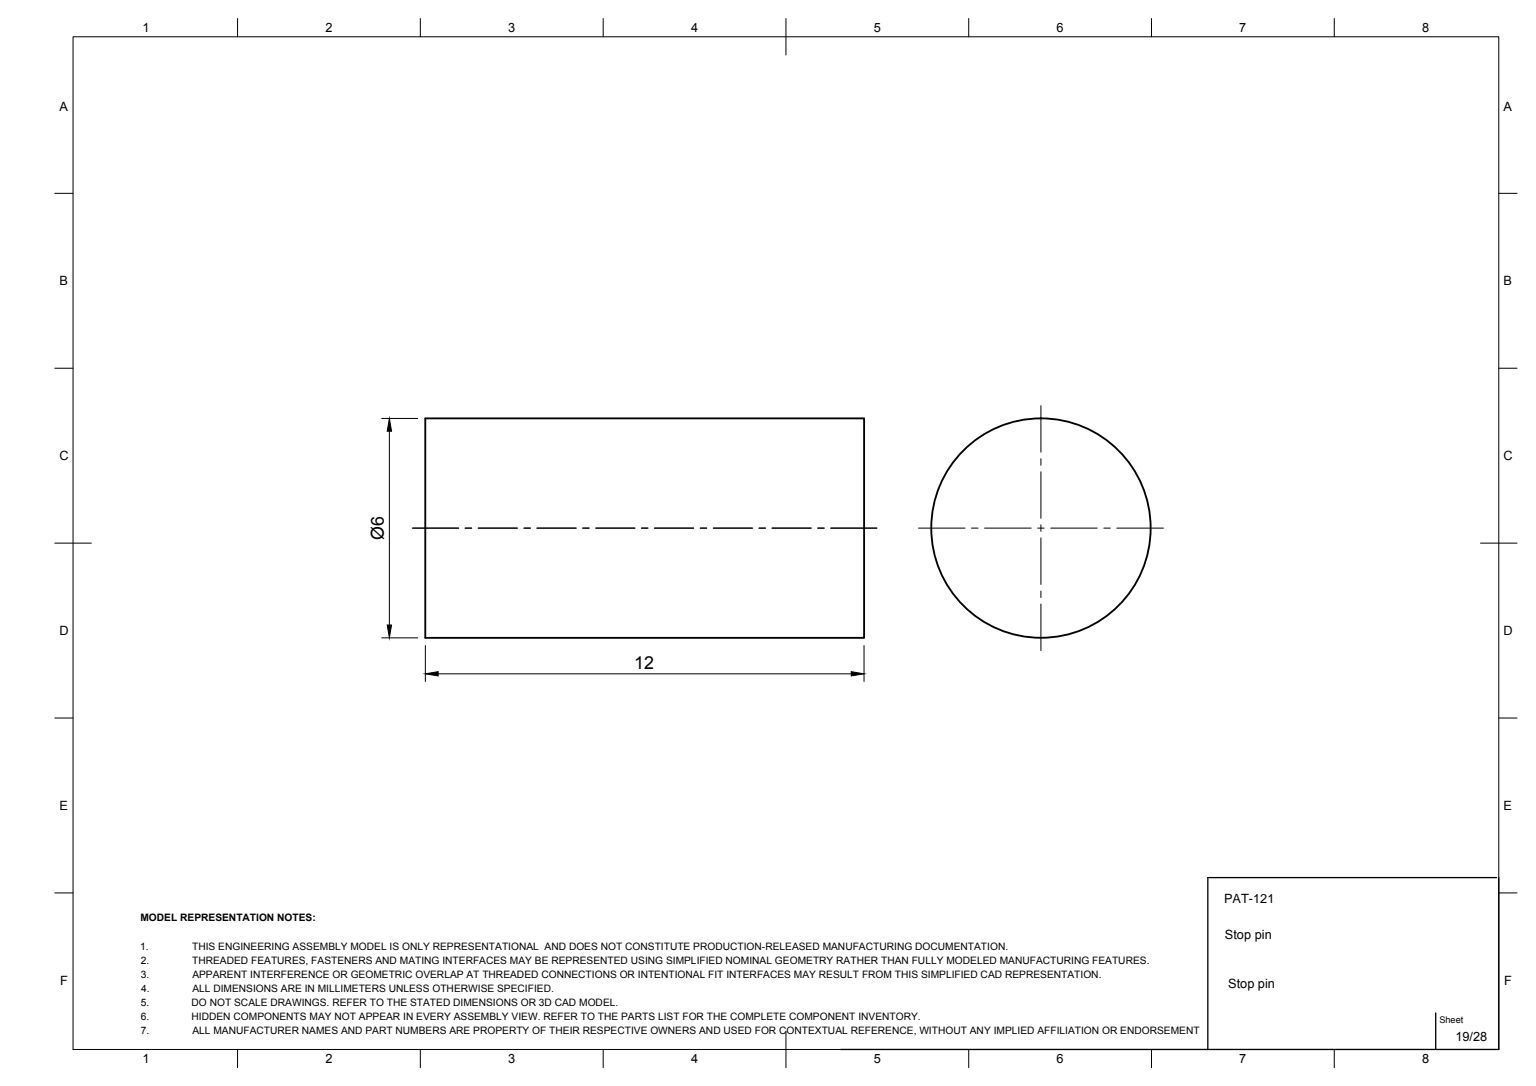
ISO-10303-21;
HEADER;
/* Generated by software containing ST-Developer
 * from STEP Tools, Inc. (www.steptools.com) 
 */

FILE_DESCRIPTION(
/* description */ ('Wall-mounted air drop station'),
/* implementation_level */ '2;1');

FILE_NAME(
/* name */ 'Stop pin.step',
/* time_stamp */ '2026-10-28T22:16:19-07:00',
/* author */ (''),
/* organization */ (''),
/* preprocessor_version */ 'ST-DEVELOPER v20.2',
/* originating_system */ 'Autodesk Translation Framework v15.17.0.0',
/* authorisation */ '');

FILE_SCHEMA (('AUTOMOTIVE_DESIGN { 1 0 10303 214 3 1 1 }'));
ENDSEC;

DATA;
#10=MECHANICAL_DESIGN_GEOMETRIC_PRESENTATION_REPRESENTATION('',(#363),#10517);
#305=SHAPE_REPRESENTATION_RELATIONSHIP('SRR','None',#10662,#334);
#334=ADVANCED_BREP_SHAPE_REPRESENTATION('',(#390),#10506);
#363=STYLED_ITEM('',(#10874),#390);
#390=MANIFOLD_SOLID_BREP('Body1',#5904);
#674=PLANE('',#6683);
#675=PLANE('',#6684);
#999=FACE_OUTER_BOUND('',#1460,.T.);
#1000=FACE_OUTER_BOUND('',#1461,.T.);
#1001=FACE_OUTER_BOUND('',#1462,.T.);
#1460=EDGE_LOOP('',(#4981,#4982,#4983,#4984));
#1461=EDGE_LOOP('',(#4985));
#1462=EDGE_LOOP('',(#4986));
#1905=LINE('',#9896,#2369);
#2369=VECTOR('',#8131,0.3);
#2699=CIRCLE('',#6681,0.3);
#2700=CIRCLE('',#6682,0.3);
#3097=VERTEX_POINT('',#9893);
#3098=VERTEX_POINT('',#9895);
#3748=EDGE_CURVE('',#3097,#3097,#2699,.T.);
#3749=EDGE_CURVE('',#3097,#3098,#1905,.T.);
#3750=EDGE_CURVE('',#3098,#3098,#2700,.T.);
#4981=ORIENTED_EDGE('',*,*,#3748,.F.);
#4982=ORIENTED_EDGE('',*,*,#3749,.T.);
#4983=ORIENTED_EDGE('',*,*,#3750,.T.);
#4984=ORIENTED_EDGE('',*,*,#3749,.F.);
#4985=ORIENTED_EDGE('',*,*,#3748,.T.);
#4986=ORIENTED_EDGE('',*,*,#3750,.F.);
#5508=CYLINDRICAL_SURFACE('',#6680,0.3);
#5772=ADVANCED_FACE('',(#999),#5508,.T.);
#5773=ADVANCED_FACE('',(#1000),#674,.T.);
#5774=ADVANCED_FACE('',(#1001),#675,.F.);
#5904=CLOSED_SHELL('',(#5772,#5773,#5774));
#6679=AXIS2_PLACEMENT_3D('',#9891,#8125,#8126);
#6680=AXIS2_PLACEMENT_3D('',#9892,#8127,#8128);
#6681=AXIS2_PLACEMENT_3D('',#9894,#8129,#8130);
#6682=AXIS2_PLACEMENT_3D('',#9897,#8132,#8133);
#6683=AXIS2_PLACEMENT_3D('',#9898,#8134,#8135);
#6684=AXIS2_PLACEMENT_3D('',#9899,#8136,#8137);
#8125=DIRECTION('axis',(0.,0.,1.));
#8126=DIRECTION('refdir',(1.,0.,0.));
#8127=DIRECTION('center_axis',(0.,0.,1.));
#8128=DIRECTION('ref_axis',(1.,0.,0.));
#8129=DIRECTION('center_axis',(0.,0.,1.));
#8130=DIRECTION('ref_axis',(1.,0.,0.));
#8131=DIRECTION('',(0.,0.,-1.));
#8132=DIRECTION('center_axis',(0.,0.,1.));
#8133=DIRECTION('ref_axis',(1.,0.,0.));
#8134=DIRECTION('center_axis',(0.,0.,1.));
#8135=DIRECTION('ref_axis',(1.,0.,0.));
#8136=DIRECTION('center_axis',(0.,0.,1.));
#8137=DIRECTION('ref_axis',(1.,0.,0.));
#9891=CARTESIAN_POINT('',(0.,0.,0.));
#9892=CARTESIAN_POINT('Origin',(3.,1.1,8.2));
#9893=CARTESIAN_POINT('',(2.7,1.1,9.4));
#9894=CARTESIAN_POINT('Origin',(3.,1.1,9.4));
#9895=CARTESIAN_POINT('',(2.7,1.1,8.2));
#9896=CARTESIAN_POINT('',(2.7,1.1,8.2));
#9897=CARTESIAN_POINT('Origin',(3.,1.1,8.2));
#9898=CARTESIAN_POINT('Origin',(3.,1.1,9.4));
#9899=CARTESIAN_POINT('Origin',(3.,1.1,8.2));
#10473=UNCERTAINTY_MEASURE_WITH_UNIT(LENGTH_MEASURE(0.001),#10518,
'DISTANCE_ACCURACY_VALUE',
'Maximum model space distance between geometric entities at asserted c
onnectivities');
#10484=UNCERTAINTY_MEASURE_WITH_UNIT(LENGTH_MEASURE(0.001),#10518,
'DISTANCE_ACCURACY_VALUE',
'Maximum model space distance between geometric entities at asserted c
onnectivities');
#10506=(
GEOMETRIC_REPRESENTATION_CONTEXT(3)
GLOBAL_UNCERTAINTY_ASSIGNED_CONTEXT((#10473))
GLOBAL_UNIT_ASSIGNED_CONTEXT((#10518,#10520,#10521))
REPRESENTATION_CONTEXT('','3D')
);
#10517=(
GEOMETRIC_REPRESENTATION_CONTEXT(3)
GLOBAL_UNCERTAINTY_ASSIGNED_CONTEXT((#10484))
GLOBAL_UNIT_ASSIGNED_CONTEXT((#10518,#10520,#10521))
REPRESENTATION_CONTEXT('','3D')
);
#10518=(
LENGTH_UNIT()
NAMED_UNIT(*)
SI_UNIT(.CENTI.,.METRE.)
);
#10520=(
NAMED_UNIT(*)
PLANE_ANGLE_UNIT()
SI_UNIT($,.RADIAN.)
);
#10521=(
NAMED_UNIT(*)
SI_UNIT($,.STERADIAN.)
SOLID_ANGLE_UNIT()
);
#10543=SHAPE_DEFINITION_REPRESENTATION(#10575,#10662);
#10575=PRODUCT_DEFINITION_SHAPE('',$,#10695);
#10662=SHAPE_REPRESENTATION('',(#6679),#10506);
#10673=PRODUCT_DEFINITION_CONTEXT('part definition',#10771,'design');
#10695=PRODUCT_DEFINITION('Stop pin','Stop pin',#10727,#10673);
#10727=PRODUCT_DEFINITION_FORMATION('',$,#10794);
#10771=APPLICATION_CONTEXT(
'Core Data for Automotive Mechanical Design Process');
#10772=PRODUCT_CONTEXT('part definition',#10771,'mechanical');
#10794=PRODUCT('Stop pin','Stop pin','Stop pin',(#10772));
#10868=COLOUR_RGB('Grey',0.48,0.52,0.57);
#10869=FILL_AREA_STYLE_COLOUR('',#10868);
#10870=FILL_AREA_STYLE('',(#10869));
#10871=SURFACE_STYLE_FILL_AREA(#10870);
#10872=SURFACE_SIDE_STYLE('',(#10871));
#10873=SURFACE_STYLE_USAGE(.BOTH.,#10872);
#10874=PRESENTATION_STYLE_ASSIGNMENT((#10873));
ENDSEC;
END-ISO-10303-21;
